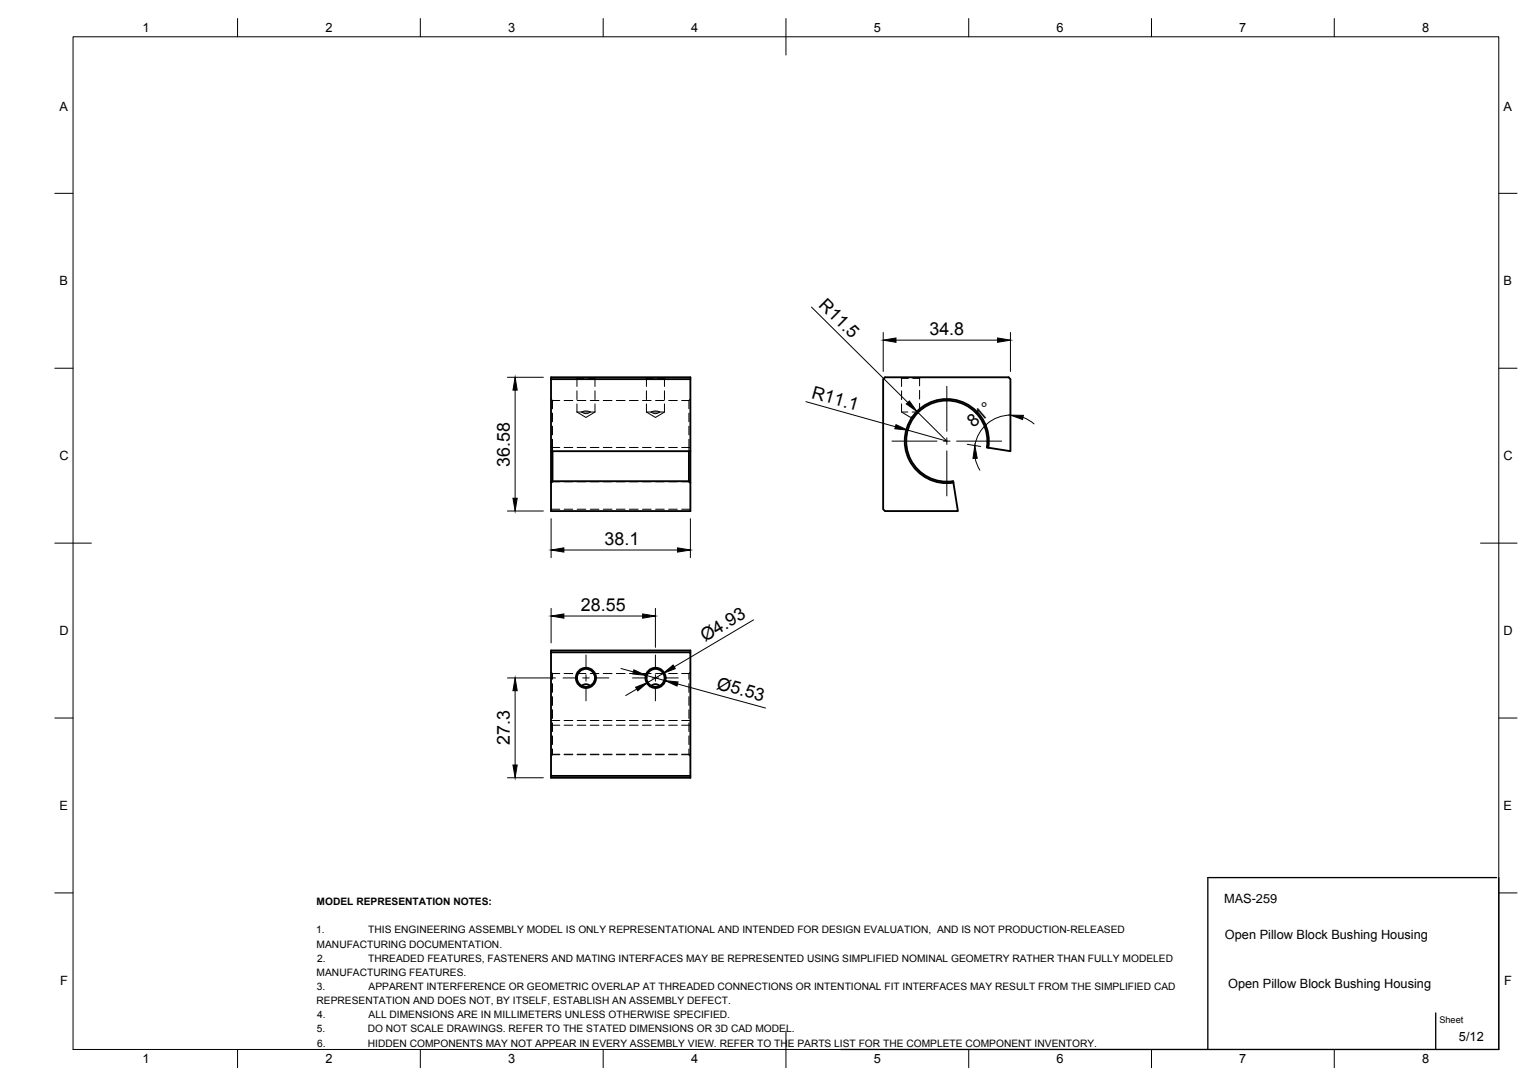
ISO-10303-21;
HEADER;
/* Generated by software containing ST-Developer
 * from STEP Tools, Inc. (www.steptools.com) 
 */

FILE_DESCRIPTION(
/* description */ (''),
/* implementation_level */ '2;1');

FILE_NAME(
/* name */ 'Open Pillow Block Bushing Housing.step',
/* time_stamp */ '2026-10-15T13:30:17-07:00',
/* author */ (''),
/* organization */ (''),
/* preprocessor_version */ 'ST-DEVELOPER v20.2',
/* originating_system */ 'Autodesk Translation Framework v15.15.0.0',
/* authorisation */ '');

FILE_SCHEMA (('AUTOMOTIVE_DESIGN { 1 0 10303 214 3 1 1 }'));
ENDSEC;

DATA;
#10=MECHANICAL_DESIGN_GEOMETRIC_PRESENTATION_REPRESENTATION('',(#1036),#71795);
#1016=SHAPE_REPRESENTATION_RELATIONSHIP('SRR','None',#72020,#1026);
#1026=ADVANCED_BREP_SHAPE_REPRESENTATION('',(#1046),#71788);
#1036=STYLED_ITEM('',(#72079),#1046);
#1046=MANIFOLD_SOLID_BREP('Body1',#13638);
#1086=CONICAL_SURFACE('',#14013,2.61400000000001,0.785398163397456);
#1087=CONICAL_SURFACE('',#14021,2.61400000000001,0.785398163397456);
#1088=CONICAL_SURFACE('',#14026,2.464,1.02974425867666);
#1089=CONICAL_SURFACE('',#14030,2.464,1.02974425867665);
#1090=CONICAL_SURFACE('',#14031,11.3,0.785398163397451);
#1091=CONICAL_SURFACE('',#14035,11.3,0.785398163397451);
#1137=B_SPLINE_CURVE_WITH_KNOTS('',3,(#19561,#19562,#19563,#19564,#19565,
#19566,#19567,#19568,#19569,#19570,#19571,#19572,#19573,#19574),
 .UNSPECIFIED.,.F.,.F.,(4,2,2,2,2,2,4),(-1.14599907215265,-1.14082829651813,
-1.08169405294193,-1.02255980936573,-0.963425565789533,-0.904291322213332,
-0.899120546578817),.UNSPECIFIED.);
#1138=B_SPLINE_CURVE_WITH_KNOTS('',3,(#19586,#19587,#19588,#19589,#19590,
#19591,#19592,#19593,#19594,#19595,#19596,#19597,#19598,#19599),
 .UNSPECIFIED.,.F.,.F.,(4,2,2,2,2,2,4),(-1.14599907215265,-1.14082829651813,
-1.08169405294193,-1.02255980936573,-0.963425565789533,-0.904291322213332,
-0.899120546578816),.UNSPECIFIED.);
#1139=B_SPLINE_CURVE_WITH_KNOTS('',3,(#19604,#19605,#19606,#19607,#19608,
#19609,#19610,#19611,#19612,#19613,#19614,#19615,#19616,#19617),
 .UNSPECIFIED.,.F.,.F.,(4,2,2,2,2,2,4),(-0.440637337632516,-0.41817718819756,
-0.36956984330978,-0.309581883490714,-0.249593923671647,-0.200986578783867,
-0.178526429348912),.UNSPECIFIED.);
#1140=B_SPLINE_CURVE_WITH_KNOTS('',3,(#19627,#19628,#19629,#19630,#19631,
#19632,#19633,#19634,#19635,#19636,#19637,#19638,#19639,#19640),
 .UNSPECIFIED.,.F.,.F.,(4,2,2,2,2,2,4),(0.787224364416541,0.851680919549612,
0.89358137447704,0.935481829404467,0.977382284331895,1.01928273925932,1.08373929439239),
 .UNSPECIFIED.);
#1545=FACE_BOUND('',#2869,.T.);
#1546=FACE_BOUND('',#2870,.T.);
#1547=FACE_BOUND('',#2876,.T.);
#1548=FACE_BOUND('',#2877,.T.);
#1613=PLANE('',#14016);
#1614=PLANE('',#14033);
#1615=PLANE('',#14034);
#1616=PLANE('',#14037);
#1617=PLANE('',#14038);
#1618=PLANE('',#14039);
#1619=PLANE('',#14040);
#1620=PLANE('',#14041);
#1621=PLANE('',#14042);
#1622=PLANE('',#14043);
#1623=PLANE('',#14044);
#2158=FACE_OUTER_BOUND('',#2867,.T.);
#2159=FACE_OUTER_BOUND('',#2868,.T.);
#2160=FACE_OUTER_BOUND('',#2871,.T.);
#2161=FACE_OUTER_BOUND('',#2872,.T.);
#2162=FACE_OUTER_BOUND('',#2873,.T.);
#2163=FACE_OUTER_BOUND('',#2874,.T.);
#2164=FACE_OUTER_BOUND('',#2875,.T.);
#2165=FACE_OUTER_BOUND('',#2878,.T.);
#2166=FACE_OUTER_BOUND('',#2879,.T.);
#2167=FACE_OUTER_BOUND('',#2880,.T.);
#2168=FACE_OUTER_BOUND('',#2881,.T.);
#2169=FACE_OUTER_BOUND('',#2882,.T.);
#2170=FACE_OUTER_BOUND('',#2883,.T.);
#2171=FACE_OUTER_BOUND('',#2884,.T.);
#2172=FACE_OUTER_BOUND('',#2885,.T.);
#2173=FACE_OUTER_BOUND('',#2886,.T.);
#2174=FACE_OUTER_BOUND('',#2887,.T.);
#2175=FACE_OUTER_BOUND('',#2888,.T.);
#2176=FACE_OUTER_BOUND('',#2889,.T.);
#2177=FACE_OUTER_BOUND('',#2890,.T.);
#2867=EDGE_LOOP('',(#9569,#9570,#9571,#9572));
#2868=EDGE_LOOP('',(#9573,#9574,#9575,#9576));
#2869=EDGE_LOOP('',(#9577));
#2870=EDGE_LOOP('',(#9578));
#2871=EDGE_LOOP('',(#9579,#9580,#9581,#9582,#9583,#9584));
#2872=EDGE_LOOP('',(#9585,#9586,#9587,#9588));
#2873=EDGE_LOOP('',(#9589,#9590,#9591,#9592,#9593,#9594));
#2874=EDGE_LOOP('',(#9595,#9596,#9597,#9598,#9599));
#2875=EDGE_LOOP('',(#9600,#9601,#9602,#9603));
#2876=EDGE_LOOP('',(#9604,#9605));
#2877=EDGE_LOOP('',(#9606,#9607));
#2878=EDGE_LOOP('',(#9608,#9609,#9610,#9611,#9612));
#2879=EDGE_LOOP('',(#9613,#9614,#9615,#9616));
#2880=EDGE_LOOP('',(#9617,#9618,#9619,#9620,#9621,#9622,#9623,#9624,#9625,
#9626));
#2881=EDGE_LOOP('',(#9627,#9628,#9629,#9630,#9631,#9632));
#2882=EDGE_LOOP('',(#9633,#9634,#9635,#9636));
#2883=EDGE_LOOP('',(#9637,#9638,#9639,#9640,#9641,#9642,#9643,#9644,#9645,
#9646));
#2884=EDGE_LOOP('',(#9647,#9648,#9649,#9650,#9651,#9652));
#2885=EDGE_LOOP('',(#9653,#9654,#9655,#9656));
#2886=EDGE_LOOP('',(#9657,#9658,#9659,#9660));
#2887=EDGE_LOOP('',(#9661,#9662,#9663,#9664));
#2888=EDGE_LOOP('',(#9665,#9666,#9667,#9668));
#2889=EDGE_LOOP('',(#9669,#9670,#9671,#9672));
#2890=EDGE_LOOP('',(#9673,#9674,#9675,#9676));
#3519=CIRCLE('',#14014,2.464);
#3520=CIRCLE('',#14015,2.76400000000001);
#3521=CIRCLE('',#14017,2.76400000000001);
#3522=CIRCLE('',#14019,2.464);
#3523=CIRCLE('',#14020,2.464);
#3524=CIRCLE('',#14022,2.464);
#3525=CIRCLE('',#14024,2.464);
#3526=CIRCLE('',#14025,2.464);
#3527=CIRCLE('',#14028,11.1);
#3528=CIRCLE('',#14029,11.1);
#3529=CIRCLE('',#14032,11.5);
#3530=CIRCLE('',#14036,11.5);
#3985=LINE('',#19542,#4896);
#3986=LINE('',#19547,#4897);
#3987=LINE('',#19549,#4898);
#3988=LINE('',#19551,#4899);
#3989=LINE('',#19552,#4900);
#3990=LINE('',#19557,#4901);
#3991=LINE('',#19579,#4902);
#3992=LINE('',#19582,#4903);
#3993=LINE('',#19603,#4904);
#3994=LINE('',#19623,#4905);
#3995=LINE('',#19626,#4906);
#3996=LINE('',#19643,#4907);
#3997=LINE('',#19646,#4908);
#3998=LINE('',#19649,#4909);
#3999=LINE('',#19652,#4910);
#4000=LINE('',#19654,#4911);
#4001=LINE('',#19655,#4912);
#4002=LINE('',#19657,#4913);
#4003=LINE('',#19659,#4914);
#4004=LINE('',#19661,#4915);
#4005=LINE('',#19663,#4916);
#4006=LINE('',#19664,#4917);
#4007=LINE('',#19667,#4918);
#4008=LINE('',#19669,#4919);
#4009=LINE('',#19670,#4920);
#4010=LINE('',#19673,#4921);
#4011=LINE('',#19677,#4922);
#4012=LINE('',#19679,#4923);
#4013=LINE('',#19681,#4924);
#4014=LINE('',#19683,#4925);
#4015=LINE('',#19684,#4926);
#4016=LINE('',#19686,#4927);
#4017=LINE('',#19687,#4928);
#4018=LINE('',#19689,#4929);
#4019=LINE('',#19691,#4930);
#4020=LINE('',#19693,#4931);
#4021=LINE('',#19695,#4932);
#4022=LINE('',#19697,#4933);
#4896=VECTOR('',#15708,2.61400000000001);
#4897=VECTOR('',#15713,10.);
#4898=VECTOR('',#15714,10.);
#4899=VECTOR('',#15715,10.);
#4900=VECTOR('',#15716,10.);
#4901=VECTOR('',#15721,2.464);
#4902=VECTOR('',#15730,2.61400000000001);
#4903=VECTOR('',#15733,2.464);
#4904=VECTOR('',#15740,2.464);
#4905=VECTOR('',#15745,10.);
#4906=VECTOR('',#15748,10.);
#4907=VECTOR('',#15751,2.464);
#4908=VECTOR('',#15754,10.);
#4909=VECTOR('',#15757,10.);
#4910=VECTOR('',#15760,10.);
#4911=VECTOR('',#15761,10.);
#4912=VECTOR('',#15762,10.);
#4913=VECTOR('',#15763,10.);
#4914=VECTOR('',#15764,10.);
#4915=VECTOR('',#15765,10.);
#4916=VECTOR('',#15766,10.);
#4917=VECTOR('',#15767,10.);
#4918=VECTOR('',#15770,10.);
#4919=VECTOR('',#15771,10.);
#4920=VECTOR('',#15772,10.);
#4921=VECTOR('',#15775,10.);
#4922=VECTOR('',#15780,10.);
#4923=VECTOR('',#15781,10.);
#4924=VECTOR('',#15782,10.);
#4925=VECTOR('',#15783,10.);
#4926=VECTOR('',#15784,10.);
#4927=VECTOR('',#15785,10.);
#4928=VECTOR('',#15786,10.);
#4929=VECTOR('',#15789,10.);
#4930=VECTOR('',#15792,10.);
#4931=VECTOR('',#15795,10.);
#4932=VECTOR('',#15798,10.);
#4933=VECTOR('',#15801,10.);
#5868=VERTEX_POINT('',#19539);
#5869=VERTEX_POINT('',#19541);
#5870=VERTEX_POINT('',#19545);
#5871=VERTEX_POINT('',#19546);
#5872=VERTEX_POINT('',#19548);
#5873=VERTEX_POINT('',#19550);
#5874=VERTEX_POINT('',#19553);
#5875=VERTEX_POINT('',#19556);
#5876=VERTEX_POINT('',#19558);
#5877=VERTEX_POINT('',#19560);
#5878=VERTEX_POINT('',#19577);
#5879=VERTEX_POINT('',#19581);
#5880=VERTEX_POINT('',#19583);
#5881=VERTEX_POINT('',#19585);
#5882=VERTEX_POINT('',#19602);
#5883=VERTEX_POINT('',#19619);
#5884=VERTEX_POINT('',#19620);
#5885=VERTEX_POINT('',#19622);
#5886=VERTEX_POINT('',#19624);
#5887=VERTEX_POINT('',#19642);
#5888=VERTEX_POINT('',#19645);
#5889=VERTEX_POINT('',#19647);
#5890=VERTEX_POINT('',#19651);
#5891=VERTEX_POINT('',#19653);
#5892=VERTEX_POINT('',#19656);
#5893=VERTEX_POINT('',#19658);
#5894=VERTEX_POINT('',#19660);
#5895=VERTEX_POINT('',#19662);
#5896=VERTEX_POINT('',#19666);
#5897=VERTEX_POINT('',#19668);
#5898=VERTEX_POINT('',#19672);
#5899=VERTEX_POINT('',#19676);
#5900=VERTEX_POINT('',#19678);
#5901=VERTEX_POINT('',#19680);
#5902=VERTEX_POINT('',#19682);
#5903=VERTEX_POINT('',#19685);
#7319=EDGE_CURVE('',#5868,#5868,#3519,.T.);
#7320=EDGE_CURVE('',#5868,#5869,#3985,.T.);
#7321=EDGE_CURVE('',#5869,#5869,#3520,.T.);
#7322=EDGE_CURVE('',#5870,#5871,#3986,.T.);
#7323=EDGE_CURVE('',#5872,#5870,#3987,.T.);
#7324=EDGE_CURVE('',#5873,#5872,#3988,.T.);
#7325=EDGE_CURVE('',#5871,#5873,#3989,.T.);
#7326=EDGE_CURVE('',#5874,#5874,#3521,.T.);
#7327=EDGE_CURVE('',#5868,#5875,#3990,.T.);
#7328=EDGE_CURVE('',#5875,#5876,#3522,.T.);
#7329=EDGE_CURVE('',#5877,#5876,#1137,.T.);
#7330=EDGE_CURVE('',#5877,#5875,#3523,.T.);
#7331=EDGE_CURVE('',#5878,#5878,#3524,.T.);
#7332=EDGE_CURVE('',#5878,#5874,#3991,.T.);
#7333=EDGE_CURVE('',#5878,#5879,#3992,.T.);
#7334=EDGE_CURVE('',#5879,#5880,#3525,.T.);
#7335=EDGE_CURVE('',#5881,#5880,#1138,.T.);
#7336=EDGE_CURVE('',#5881,#5879,#3526,.T.);
#7337=EDGE_CURVE('',#5882,#5875,#3993,.T.);
#7338=EDGE_CURVE('',#5876,#5877,#1139,.T.);
#7339=EDGE_CURVE('',#5883,#5884,#3527,.T.);
#7340=EDGE_CURVE('',#5885,#5883,#3994,.T.);
#7341=EDGE_CURVE('',#5886,#5885,#3528,.T.);
#7342=EDGE_CURVE('',#5884,#5886,#3995,.T.);
#7343=EDGE_CURVE('',#5880,#5881,#1140,.T.);
#7344=EDGE_CURVE('',#5887,#5879,#3996,.T.);
#7345=EDGE_CURVE('',#5884,#5888,#3997,.T.);
#7346=EDGE_CURVE('',#5888,#5889,#3529,.T.);
#7347=EDGE_CURVE('',#5889,#5883,#3998,.T.);
#7348=EDGE_CURVE('',#5888,#5890,#3999,.T.);
#7349=EDGE_CURVE('',#5890,#5891,#4000,.T.);
#7350=EDGE_CURVE('',#5871,#5891,#4001,.T.);
#7351=EDGE_CURVE('',#5892,#5873,#4002,.T.);
#7352=EDGE_CURVE('',#5892,#5893,#4003,.T.);
#7353=EDGE_CURVE('',#5894,#5893,#4004,.T.);
#7354=EDGE_CURVE('',#5894,#5895,#4005,.T.);
#7355=EDGE_CURVE('',#5895,#5889,#4006,.T.);
#7356=EDGE_CURVE('',#5896,#5886,#4007,.T.);
#7357=EDGE_CURVE('',#5897,#5896,#4008,.T.);
#7358=EDGE_CURVE('',#5897,#5890,#4009,.T.);
#7359=EDGE_CURVE('',#5885,#5898,#4010,.T.);
#7360=EDGE_CURVE('',#5898,#5896,#3530,.T.);
#7361=EDGE_CURVE('',#5898,#5899,#4011,.T.);
#7362=EDGE_CURVE('',#5899,#5900,#4012,.T.);
#7363=EDGE_CURVE('',#5901,#5900,#4013,.T.);
#7364=EDGE_CURVE('',#5901,#5902,#4014,.T.);
#7365=EDGE_CURVE('',#5872,#5902,#4015,.T.);
#7366=EDGE_CURVE('',#5903,#5870,#4016,.T.);
#7367=EDGE_CURVE('',#5903,#5897,#4017,.T.);
#7368=EDGE_CURVE('',#5899,#5895,#4018,.T.);
#7369=EDGE_CURVE('',#5891,#5903,#4019,.T.);
#7370=EDGE_CURVE('',#5902,#5892,#4020,.T.);
#7371=EDGE_CURVE('',#5893,#5901,#4021,.T.);
#7372=EDGE_CURVE('',#5900,#5894,#4022,.T.);
#9569=ORIENTED_EDGE('',*,*,#7319,.T.);
#9570=ORIENTED_EDGE('',*,*,#7320,.T.);
#9571=ORIENTED_EDGE('',*,*,#7321,.T.);
#9572=ORIENTED_EDGE('',*,*,#7320,.F.);
#9573=ORIENTED_EDGE('',*,*,#7322,.F.);
#9574=ORIENTED_EDGE('',*,*,#7323,.F.);
#9575=ORIENTED_EDGE('',*,*,#7324,.F.);
#9576=ORIENTED_EDGE('',*,*,#7325,.F.);
#9577=ORIENTED_EDGE('',*,*,#7326,.F.);
#9578=ORIENTED_EDGE('',*,*,#7321,.F.);
#9579=ORIENTED_EDGE('',*,*,#7319,.F.);
#9580=ORIENTED_EDGE('',*,*,#7327,.T.);
#9581=ORIENTED_EDGE('',*,*,#7328,.T.);
#9582=ORIENTED_EDGE('',*,*,#7329,.F.);
#9583=ORIENTED_EDGE('',*,*,#7330,.T.);
#9584=ORIENTED_EDGE('',*,*,#7327,.F.);
#9585=ORIENTED_EDGE('',*,*,#7331,.T.);
#9586=ORIENTED_EDGE('',*,*,#7332,.T.);
#9587=ORIENTED_EDGE('',*,*,#7326,.T.);
#9588=ORIENTED_EDGE('',*,*,#7332,.F.);
#9589=ORIENTED_EDGE('',*,*,#7331,.F.);
#9590=ORIENTED_EDGE('',*,*,#7333,.T.);
#9591=ORIENTED_EDGE('',*,*,#7334,.T.);
#9592=ORIENTED_EDGE('',*,*,#7335,.F.);
#9593=ORIENTED_EDGE('',*,*,#7336,.T.);
#9594=ORIENTED_EDGE('',*,*,#7333,.F.);
#9595=ORIENTED_EDGE('',*,*,#7337,.T.);
#9596=ORIENTED_EDGE('',*,*,#7330,.F.);
#9597=ORIENTED_EDGE('',*,*,#7338,.F.);
#9598=ORIENTED_EDGE('',*,*,#7328,.F.);
#9599=ORIENTED_EDGE('',*,*,#7337,.F.);
#9600=ORIENTED_EDGE('',*,*,#7339,.F.);
#9601=ORIENTED_EDGE('',*,*,#7340,.F.);
#9602=ORIENTED_EDGE('',*,*,#7341,.F.);
#9603=ORIENTED_EDGE('',*,*,#7342,.F.);
#9604=ORIENTED_EDGE('',*,*,#7343,.T.);
#9605=ORIENTED_EDGE('',*,*,#7335,.T.);
#9606=ORIENTED_EDGE('',*,*,#7338,.T.);
#9607=ORIENTED_EDGE('',*,*,#7329,.T.);
#9608=ORIENTED_EDGE('',*,*,#7344,.T.);
#9609=ORIENTED_EDGE('',*,*,#7336,.F.);
#9610=ORIENTED_EDGE('',*,*,#7343,.F.);
#9611=ORIENTED_EDGE('',*,*,#7334,.F.);
#9612=ORIENTED_EDGE('',*,*,#7344,.F.);
#9613=ORIENTED_EDGE('',*,*,#7345,.T.);
#9614=ORIENTED_EDGE('',*,*,#7346,.T.);
#9615=ORIENTED_EDGE('',*,*,#7347,.T.);
#9616=ORIENTED_EDGE('',*,*,#7339,.T.);
#9617=ORIENTED_EDGE('',*,*,#7346,.F.);
#9618=ORIENTED_EDGE('',*,*,#7348,.T.);
#9619=ORIENTED_EDGE('',*,*,#7349,.T.);
#9620=ORIENTED_EDGE('',*,*,#7350,.F.);
#9621=ORIENTED_EDGE('',*,*,#7325,.T.);
#9622=ORIENTED_EDGE('',*,*,#7351,.F.);
#9623=ORIENTED_EDGE('',*,*,#7352,.T.);
#9624=ORIENTED_EDGE('',*,*,#7353,.F.);
#9625=ORIENTED_EDGE('',*,*,#7354,.T.);
#9626=ORIENTED_EDGE('',*,*,#7355,.T.);
#9627=ORIENTED_EDGE('',*,*,#7345,.F.);
#9628=ORIENTED_EDGE('',*,*,#7342,.T.);
#9629=ORIENTED_EDGE('',*,*,#7356,.F.);
#9630=ORIENTED_EDGE('',*,*,#7357,.F.);
#9631=ORIENTED_EDGE('',*,*,#7358,.T.);
#9632=ORIENTED_EDGE('',*,*,#7348,.F.);
#9633=ORIENTED_EDGE('',*,*,#7359,.T.);
#9634=ORIENTED_EDGE('',*,*,#7360,.T.);
#9635=ORIENTED_EDGE('',*,*,#7356,.T.);
#9636=ORIENTED_EDGE('',*,*,#7341,.T.);
#9637=ORIENTED_EDGE('',*,*,#7360,.F.);
#9638=ORIENTED_EDGE('',*,*,#7361,.T.);
#9639=ORIENTED_EDGE('',*,*,#7362,.T.);
#9640=ORIENTED_EDGE('',*,*,#7363,.F.);
#9641=ORIENTED_EDGE('',*,*,#7364,.T.);
#9642=ORIENTED_EDGE('',*,*,#7365,.F.);
#9643=ORIENTED_EDGE('',*,*,#7323,.T.);
#9644=ORIENTED_EDGE('',*,*,#7366,.F.);
#9645=ORIENTED_EDGE('',*,*,#7367,.T.);
#9646=ORIENTED_EDGE('',*,*,#7357,.T.);
#9647=ORIENTED_EDGE('',*,*,#7347,.F.);
#9648=ORIENTED_EDGE('',*,*,#7355,.F.);
#9649=ORIENTED_EDGE('',*,*,#7368,.F.);
#9650=ORIENTED_EDGE('',*,*,#7361,.F.);
#9651=ORIENTED_EDGE('',*,*,#7359,.F.);
#9652=ORIENTED_EDGE('',*,*,#7340,.T.);
#9653=ORIENTED_EDGE('',*,*,#7350,.T.);
#9654=ORIENTED_EDGE('',*,*,#7369,.T.);
#9655=ORIENTED_EDGE('',*,*,#7366,.T.);
#9656=ORIENTED_EDGE('',*,*,#7322,.T.);
#9657=ORIENTED_EDGE('',*,*,#7351,.T.);
#9658=ORIENTED_EDGE('',*,*,#7324,.T.);
#9659=ORIENTED_EDGE('',*,*,#7365,.T.);
#9660=ORIENTED_EDGE('',*,*,#7370,.T.);
#9661=ORIENTED_EDGE('',*,*,#7370,.F.);
#9662=ORIENTED_EDGE('',*,*,#7364,.F.);
#9663=ORIENTED_EDGE('',*,*,#7371,.F.);
#9664=ORIENTED_EDGE('',*,*,#7352,.F.);
#9665=ORIENTED_EDGE('',*,*,#7353,.T.);
#9666=ORIENTED_EDGE('',*,*,#7371,.T.);
#9667=ORIENTED_EDGE('',*,*,#7363,.T.);
#9668=ORIENTED_EDGE('',*,*,#7372,.T.);
#9669=ORIENTED_EDGE('',*,*,#7372,.F.);
#9670=ORIENTED_EDGE('',*,*,#7362,.F.);
#9671=ORIENTED_EDGE('',*,*,#7368,.T.);
#9672=ORIENTED_EDGE('',*,*,#7354,.F.);
#9673=ORIENTED_EDGE('',*,*,#7369,.F.);
#9674=ORIENTED_EDGE('',*,*,#7349,.F.);
#9675=ORIENTED_EDGE('',*,*,#7358,.F.);
#9676=ORIENTED_EDGE('',*,*,#7367,.F.);
#12911=CYLINDRICAL_SURFACE('',#14018,2.464);
#12912=CYLINDRICAL_SURFACE('',#14023,2.464);
#12913=CYLINDRICAL_SURFACE('',#14027,11.1);
#13118=ADVANCED_FACE('',(#2158),#1086,.F.);
#13119=ADVANCED_FACE('',(#2159,#1545,#1546),#1613,.T.);
#13120=ADVANCED_FACE('',(#2160),#12911,.F.);
#13121=ADVANCED_FACE('',(#2161),#1087,.F.);
#13122=ADVANCED_FACE('',(#2162),#12912,.F.);
#13123=ADVANCED_FACE('',(#2163),#1088,.F.);
#13124=ADVANCED_FACE('',(#2164,#1547,#1548),#12913,.F.);
#13125=ADVANCED_FACE('',(#2165),#1089,.F.);
#13126=ADVANCED_FACE('',(#2166),#1090,.F.);
#13127=ADVANCED_FACE('',(#2167),#1614,.T.);
#13128=ADVANCED_FACE('',(#2168),#1615,.T.);
#13129=ADVANCED_FACE('',(#2169),#1091,.F.);
#13130=ADVANCED_FACE('',(#2170),#1616,.F.);
#13131=ADVANCED_FACE('',(#2171),#1617,.T.);
#13132=ADVANCED_FACE('',(#2172),#1618,.T.);
#13133=ADVANCED_FACE('',(#2173),#1619,.T.);
#13134=ADVANCED_FACE('',(#2174),#1620,.T.);
#13135=ADVANCED_FACE('',(#2175),#1621,.T.);
#13136=ADVANCED_FACE('',(#2176),#1622,.T.);
#13137=ADVANCED_FACE('',(#2177),#1623,.T.);
#13638=CLOSED_SHELL('',(#13118,#13119,#13120,#13121,#13122,#13123,#13124,
#13125,#13126,#13127,#13128,#13129,#13130,#13131,#13132,#13133,#13134,#13135,
#13136,#13137));
#14012=AXIS2_PLACEMENT_3D('',#19537,#15702,#15703);
#14013=AXIS2_PLACEMENT_3D('',#19538,#15704,#15705);
#14014=AXIS2_PLACEMENT_3D('',#19540,#15706,#15707);
#14015=AXIS2_PLACEMENT_3D('',#19543,#15709,#15710);
#14016=AXIS2_PLACEMENT_3D('',#19544,#15711,#15712);
#14017=AXIS2_PLACEMENT_3D('',#19554,#15717,#15718);
#14018=AXIS2_PLACEMENT_3D('',#19555,#15719,#15720);
#14019=AXIS2_PLACEMENT_3D('',#19559,#15722,#15723);
#14020=AXIS2_PLACEMENT_3D('',#19575,#15724,#15725);
#14021=AXIS2_PLACEMENT_3D('',#19576,#15726,#15727);
#14022=AXIS2_PLACEMENT_3D('',#19578,#15728,#15729);
#14023=AXIS2_PLACEMENT_3D('',#19580,#15731,#15732);
#14024=AXIS2_PLACEMENT_3D('',#19584,#15734,#15735);
#14025=AXIS2_PLACEMENT_3D('',#19600,#15736,#15737);
#14026=AXIS2_PLACEMENT_3D('',#19601,#15738,#15739);
#14027=AXIS2_PLACEMENT_3D('',#19618,#15741,#15742);
#14028=AXIS2_PLACEMENT_3D('',#19621,#15743,#15744);
#14029=AXIS2_PLACEMENT_3D('',#19625,#15746,#15747);
#14030=AXIS2_PLACEMENT_3D('',#19641,#15749,#15750);
#14031=AXIS2_PLACEMENT_3D('',#19644,#15752,#15753);
#14032=AXIS2_PLACEMENT_3D('',#19648,#15755,#15756);
#14033=AXIS2_PLACEMENT_3D('',#19650,#15758,#15759);
#14034=AXIS2_PLACEMENT_3D('',#19665,#15768,#15769);
#14035=AXIS2_PLACEMENT_3D('',#19671,#15773,#15774);
#14036=AXIS2_PLACEMENT_3D('',#19674,#15776,#15777);
#14037=AXIS2_PLACEMENT_3D('',#19675,#15778,#15779);
#14038=AXIS2_PLACEMENT_3D('',#19688,#15787,#15788);
#14039=AXIS2_PLACEMENT_3D('',#19690,#15790,#15791);
#14040=AXIS2_PLACEMENT_3D('',#19692,#15793,#15794);
#14041=AXIS2_PLACEMENT_3D('',#19694,#15796,#15797);
#14042=AXIS2_PLACEMENT_3D('',#19696,#15799,#15800);
#14043=AXIS2_PLACEMENT_3D('',#19698,#15802,#15803);
#14044=AXIS2_PLACEMENT_3D('',#19699,#15804,#15805);
#15702=DIRECTION('axis',(0.,0.,1.));
#15703=DIRECTION('refdir',(1.,0.,0.));
#15704=DIRECTION('center_axis',(0.,1.,0.));
#15705=DIRECTION('ref_axis',(1.,0.,0.));
#15706=DIRECTION('center_axis',(0.,-1.,0.));
#15707=DIRECTION('ref_axis',(1.,0.,0.));
#15708=DIRECTION('',(-0.707106781186553,0.707106781186542,8.659560562355E-17));
#15709=DIRECTION('center_axis',(0.,1.,0.));
#15710=DIRECTION('ref_axis',(1.,0.,0.));
#15711=DIRECTION('center_axis',(0.,1.,0.));
#15712=DIRECTION('ref_axis',(0.,0.,1.));
#15713=DIRECTION('',(1.,0.,0.));
#15714=DIRECTION('',(0.,0.,-1.));
#15715=DIRECTION('',(-1.,0.,0.));
#15716=DIRECTION('',(0.,0.,1.));
#15717=DIRECTION('center_axis',(0.,1.,0.));
#15718=DIRECTION('ref_axis',(1.,0.,0.));
#15719=DIRECTION('center_axis',(0.,-1.,0.));
#15720=DIRECTION('ref_axis',(1.,0.,0.));
#15721=DIRECTION('',(0.,-1.,0.));
#15722=DIRECTION('center_axis',(0.,-1.,0.));
#15723=DIRECTION('ref_axis',(1.,0.,0.));
#15724=DIRECTION('center_axis',(0.,-1.,0.));
#15725=DIRECTION('ref_axis',(1.,0.,0.));
#15726=DIRECTION('center_axis',(0.,1.,0.));
#15727=DIRECTION('ref_axis',(1.,0.,0.));
#15728=DIRECTION('center_axis',(0.,-1.,0.));
#15729=DIRECTION('ref_axis',(1.,0.,0.));
#15730=DIRECTION('',(-0.707106781186553,0.707106781186542,8.659560562355E-17));
#15731=DIRECTION('center_axis',(0.,-1.,0.));
#15732=DIRECTION('ref_axis',(1.,0.,0.));
#15733=DIRECTION('',(0.,-1.,0.));
#15734=DIRECTION('center_axis',(0.,-1.,0.));
#15735=DIRECTION('ref_axis',(1.,0.,0.));
#15736=DIRECTION('center_axis',(0.,-1.,0.));
#15737=DIRECTION('ref_axis',(1.,0.,0.));
#15738=DIRECTION('center_axis',(0.,1.,0.));
#15739=DIRECTION('ref_axis',(1.,0.,0.));
#15740=DIRECTION('',(-0.857167300702115,0.515038074910049,1.04972719113862E-16));
#15741=DIRECTION('center_axis',(1.,0.,0.));
#15742=DIRECTION('ref_axis',(0.,0.707106781186547,0.707106781186547));
#15743=DIRECTION('center_axis',(-1.,0.,0.));
#15744=DIRECTION('ref_axis',(0.,0.,1.));
#15745=DIRECTION('',(1.,0.,0.));
#15746=DIRECTION('center_axis',(1.,0.,0.));
#15747=DIRECTION('ref_axis',(0.,0.,1.));
#15748=DIRECTION('',(-1.,0.,0.));
#15749=DIRECTION('center_axis',(0.,1.,0.));
#15750=DIRECTION('ref_axis',(1.,0.,0.));
#15751=DIRECTION('',(-0.85716730070211,0.515038074910058,1.04972719113862E-16));
#15752=DIRECTION('center_axis',(1.,0.,0.));
#15753=DIRECTION('ref_axis',(0.,0.707106781186547,0.707106781186548));
#15754=DIRECTION('',(0.707106781186546,-0.110615871041237,-0.698401123333712));
#15755=DIRECTION('center_axis',(1.,0.,0.));
#15756=DIRECTION('ref_axis',(0.,0.,1.));
#15757=DIRECTION('',(-0.707106781186546,0.698401123333712,0.110615871041237));
#15758=DIRECTION('center_axis',(1.,0.,0.));
#15759=DIRECTION('ref_axis',(0.,0.,-1.));
#15760=DIRECTION('',(0.,-0.156434465040231,-0.987688340595138));
#15761=DIRECTION('',(0.,1.,0.));
#15762=DIRECTION('',(0.,-0.707106781186547,-0.707106781186547));
#15763=DIRECTION('',(0.,0.707106781186547,-0.707106781186547));
#15764=DIRECTION('',(0.,-1.,0.));
#15765=DIRECTION('',(0.,0.707106781186543,0.707106781186552));
#15766=DIRECTION('',(0.,0.,-1.));
#15767=DIRECTION('',(0.,0.987688340595138,0.156434465040231));
#15768=DIRECTION('center_axis',(0.,-0.987688340595138,0.156434465040231));
#15769=DIRECTION('ref_axis',(0.,-0.156434465040231,-0.987688340595138));
#15770=DIRECTION('',(0.707106781186546,0.110615871041237,0.698401123333712));
#15771=DIRECTION('',(0.,0.156434465040231,0.987688340595138));
#15772=DIRECTION('',(1.,0.,0.));
#15773=DIRECTION('center_axis',(-1.,0.,0.));
#15774=DIRECTION('ref_axis',(0.,0.707106781186547,0.707106781186548));
#15775=DIRECTION('',(-0.707106781186546,-0.698401123333712,-0.110615871041237));
#15776=DIRECTION('center_axis',(-1.,0.,0.));
#15777=DIRECTION('ref_axis',(0.,0.,1.));
#15778=DIRECTION('center_axis',(1.,0.,0.));
#15779=DIRECTION('ref_axis',(0.,0.,-1.));
#15780=DIRECTION('',(0.,-0.987688340595138,-0.156434465040231));
#15781=DIRECTION('',(0.,0.,1.));
#15782=DIRECTION('',(0.,-0.707106781186543,-0.707106781186552));
#15783=DIRECTION('',(0.,1.,0.));
#15784=DIRECTION('',(0.,-0.707106781186547,0.707106781186547));
#15785=DIRECTION('',(0.,0.707106781186547,0.707106781186547));
#15786=DIRECTION('',(0.,-1.,0.));
#15787=DIRECTION('center_axis',(0.,0.156434465040231,-0.987688340595138));
#15788=DIRECTION('ref_axis',(0.,0.987688340595138,0.156434465040231));
#15789=DIRECTION('',(1.,0.,0.));
#15790=DIRECTION('center_axis',(0.,0.707106781186548,-0.707106781186548));
#15791=DIRECTION('ref_axis',(-1.,0.,0.));
#15792=DIRECTION('',(-1.,0.,0.));
#15793=DIRECTION('center_axis',(0.,0.707106781186548,0.707106781186548));
#15794=DIRECTION('ref_axis',(1.,0.,0.));
#15795=DIRECTION('',(1.,0.,0.));
#15796=DIRECTION('center_axis',(0.,0.,1.));
#15797=DIRECTION('ref_axis',(0.,-1.,0.));
#15798=DIRECTION('',(-1.,0.,0.));
#15799=DIRECTION('center_axis',(0.,-0.707106781186552,0.707106781186543));
#15800=DIRECTION('ref_axis',(1.,0.,0.));
#15801=DIRECTION('',(1.,0.,0.));
#15802=DIRECTION('center_axis',(0.,-1.,0.));
#15803=DIRECTION('ref_axis',(0.,0.,-1.));
#15804=DIRECTION('center_axis',(0.,0.,-1.));
#15805=DIRECTION('ref_axis',(0.,1.,0.));
#19537=CARTESIAN_POINT('',(0.,0.,0.));
#19538=CARTESIAN_POINT('Origin',(61.4,39.5248,48.));
#19539=CARTESIAN_POINT('',(58.936,39.3748,48.));
#19540=CARTESIAN_POINT('Origin',(61.4,39.3748,48.));
#19541=CARTESIAN_POINT('',(58.636,39.6748,48.));
#19542=CARTESIAN_POINT('',(58.786,39.5248,48.));
#19543=CARTESIAN_POINT('Origin',(61.4,39.6748,48.));
#19544=CARTESIAN_POINT('Origin',(32.85,39.6748,20.7));
#19545=CARTESIAN_POINT('',(32.85,39.6748,21.2));
#19546=CARTESIAN_POINT('',(70.95,39.6748,21.2));
#19547=CARTESIAN_POINT('',(32.85,39.6748,21.2));
#19548=CARTESIAN_POINT('',(32.85,39.6748,54.999));
#19549=CARTESIAN_POINT('',(32.85,39.6748,55.499));
#19550=CARTESIAN_POINT('',(70.95,39.6748,54.999));
#19551=CARTESIAN_POINT('',(32.85,39.6748,54.999));
#19552=CARTESIAN_POINT('',(70.95,39.6748,55.499));
#19553=CARTESIAN_POINT('',(39.636,39.6748,48.));
#19554=CARTESIAN_POINT('Origin',(42.4,39.6748,48.));
#19555=CARTESIAN_POINT('Origin',(61.4,39.6748,48.));
#19556=CARTESIAN_POINT('',(58.936,30.1748,48.));
#19557=CARTESIAN_POINT('',(58.936,39.6748,48.));
#19558=CARTESIAN_POINT('',(60.2023331707725,30.1748,45.8466560501935));
#19559=CARTESIAN_POINT('Origin',(61.4,30.1748,48.));
#19560=CARTESIAN_POINT('',(62.5976668292275,30.1748,45.8466560501935));
#19561=CARTESIAN_POINT('Ctrl Pts',(62.5976668292275,30.1748,45.8466560501935));
#19562=CARTESIAN_POINT('Ctrl Pts',(62.5839393404939,30.1822399802705,45.8390209680664));
#19563=CARTESIAN_POINT('Ctrl Pts',(62.5701440730763,30.1895277245944,45.8315201115594));
#19564=CARTESIAN_POINT('Ctrl Pts',(62.3978378742979,30.2782518989111,45.7399529520181));
#19565=CARTESIAN_POINT('Ctrl Pts',(62.2093398392196,30.3494894405534,45.6635629490944));
#19566=CARTESIAN_POINT('Ctrl Pts',(61.8090152862429,30.4433961447374,45.5614192720633));
#19567=CARTESIAN_POINT('Ctrl Pts',(61.597114145254,30.4661106047668,45.536));
#19568=CARTESIAN_POINT('Ctrl Pts',(61.202885854746,30.4661106047668,45.536));
#19569=CARTESIAN_POINT('Ctrl Pts',(60.9909847137571,30.4433961447374,45.5614192720633));
#19570=CARTESIAN_POINT('Ctrl Pts',(60.5906601607804,30.3494894405534,45.6635629490944));
#19571=CARTESIAN_POINT('Ctrl Pts',(60.4021621257021,30.2782518989111,45.7399529520181));
#19572=CARTESIAN_POINT('Ctrl Pts',(60.2298559269237,30.1895277245944,45.8315201115594));
#19573=CARTESIAN_POINT('Ctrl Pts',(60.2160606595061,30.1822399802704,45.8390209680664));
#19574=CARTESIAN_POINT('Ctrl Pts',(60.2023331707725,30.1748,45.8466560501935));
#19575=CARTESIAN_POINT('Origin',(61.4,30.1748,48.));
#19576=CARTESIAN_POINT('Origin',(42.4,39.5248,48.));
#19577=CARTESIAN_POINT('',(39.936,39.3748,48.));
#19578=CARTESIAN_POINT('Origin',(42.4,39.3748,48.));
#19579=CARTESIAN_POINT('',(39.786,39.5248,48.));
#19580=CARTESIAN_POINT('Origin',(42.4,39.6748,48.));
#19581=CARTESIAN_POINT('',(39.936,30.1748,48.));
#19582=CARTESIAN_POINT('',(39.936,39.6748,48.));
#19583=CARTESIAN_POINT('',(41.2023331707725,30.1748,45.8466560501935));
#19584=CARTESIAN_POINT('Origin',(42.4,30.1748,48.));
#19585=CARTESIAN_POINT('',(43.5976668292275,30.1748,45.8466560501935));
#19586=CARTESIAN_POINT('Ctrl Pts',(43.5976668292275,30.1748,45.8466560501935));
#19587=CARTESIAN_POINT('Ctrl Pts',(43.5839393404939,30.1822399802704,45.8390209680664));
#19588=CARTESIAN_POINT('Ctrl Pts',(43.5701440730763,30.1895277245944,45.8315201115594));
#19589=CARTESIAN_POINT('Ctrl Pts',(43.3978378742979,30.2782518989111,45.7399529520181));
#19590=CARTESIAN_POINT('Ctrl Pts',(43.2093398392196,30.3494894405534,45.6635629490944));
#19591=CARTESIAN_POINT('Ctrl Pts',(42.8090152862429,30.4433961447374,45.5614192720633));
#19592=CARTESIAN_POINT('Ctrl Pts',(42.597114145254,30.4661106047668,45.536));
#19593=CARTESIAN_POINT('Ctrl Pts',(42.202885854746,30.4661106047668,45.536));
#19594=CARTESIAN_POINT('Ctrl Pts',(41.9909847137571,30.4433961447374,45.5614192720633));
#19595=CARTESIAN_POINT('Ctrl Pts',(41.5906601607804,30.3494894405534,45.6635629490944));
#19596=CARTESIAN_POINT('Ctrl Pts',(41.4021621257021,30.2782518989111,45.7399529520181));
#19597=CARTESIAN_POINT('Ctrl Pts',(41.2298559269237,30.1895277245944,45.8315201115594));
#19598=CARTESIAN_POINT('Ctrl Pts',(41.216060659506,30.1822399802704,45.8390209680664));
#19599=CARTESIAN_POINT('Ctrl Pts',(41.2023331707725,30.1748,45.8466560501935));
#19600=CARTESIAN_POINT('Origin',(42.4,30.1748,48.));
#19601=CARTESIAN_POINT('Origin',(61.4,30.1748,48.));
#19602=CARTESIAN_POINT('',(61.4,28.6942794347161,48.));
#19603=CARTESIAN_POINT('',(58.936,30.1748,48.));
#19604=CARTESIAN_POINT('Ctrl Pts',(60.2023331707725,30.1748,45.8466560501935));
#19605=CARTESIAN_POINT('Ctrl Pts',(60.2597361109102,30.1384432612634,45.8839661875916));
#19606=CARTESIAN_POINT('Ctrl Pts',(60.3174608135473,30.1032893210344,45.9195148810763));
#19607=CARTESIAN_POINT('Ctrl Pts',(60.5005858709669,29.9969713807309,46.0257192203701));
#19608=CARTESIAN_POINT('Ctrl Pts',(60.6580928550894,29.9150369491545,46.1049725011069));
#19609=CARTESIAN_POINT('Ctrl Pts',(60.9740384574878,29.7867651942036,46.2264525494457));
#19610=CARTESIAN_POINT('Ctrl Pts',(61.2000401339365,29.7272527548782,46.2808436974387));
#19611=CARTESIAN_POINT('Ctrl Pts',(61.5999598660636,29.7272527548782,46.2808436974387));
#19612=CARTESIAN_POINT('Ctrl Pts',(61.8259615425122,29.7867651942036,46.2264525494457));
#19613=CARTESIAN_POINT('Ctrl Pts',(62.1419071449106,29.9150369491545,46.1049725011069));
#19614=CARTESIAN_POINT('Ctrl Pts',(62.2994141290331,29.9969713807309,46.0257192203701));
#19615=CARTESIAN_POINT('Ctrl Pts',(62.4825391864527,30.1032893210343,45.9195148810763));
#19616=CARTESIAN_POINT('Ctrl Pts',(62.5402638890898,30.1384432612634,45.8839661875916));
#19617=CARTESIAN_POINT('Ctrl Pts',(62.5976668292275,30.1748,45.8466560501935));
#19618=CARTESIAN_POINT('Origin',(32.85,22.225,38.1));
#19619=CARTESIAN_POINT('',(70.55,11.261659419394,36.3635774380534));
#19620=CARTESIAN_POINT('',(70.55,20.4885774380534,27.136659419394));
#19621=CARTESIAN_POINT('Origin',(70.55,22.225,38.1));
#19622=CARTESIAN_POINT('',(33.25,11.261659419394,36.3635774380534));
#19623=CARTESIAN_POINT('',(32.85,11.261659419394,36.3635774380534));
#19624=CARTESIAN_POINT('',(33.25,20.4885774380534,27.136659419394));
#19625=CARTESIAN_POINT('Origin',(33.25,22.225,38.1));
#19626=CARTESIAN_POINT('',(32.85,20.4885774380534,27.136659419394));
#19627=CARTESIAN_POINT('Ctrl Pts',(41.2023331707725,30.1748,45.8466560501935));
#19628=CARTESIAN_POINT('Ctrl Pts',(41.3584359963022,30.0759306802366,45.9481180633722));
#19629=CARTESIAN_POINT('Ctrl Pts',(41.5172853281954,29.9848847225031,46.0375998429581));
#19630=CARTESIAN_POINT('Ctrl Pts',(41.7909111977588,29.8583912347539,46.1589138702689));
#19631=CARTESIAN_POINT('Ctrl Pts',(41.9011722141917,29.8148256477821,46.1997866389185));
#19632=CARTESIAN_POINT('Ctrl Pts',(42.1359436639152,29.7493650522022,46.2606327740154));
#19633=CARTESIAN_POINT('Ctrl Pts',(42.2603318169086,29.7272527548782,46.2808436974387));
#19634=CARTESIAN_POINT('Ctrl Pts',(42.5396681830914,29.7272527548782,46.2808436974387));
#19635=CARTESIAN_POINT('Ctrl Pts',(42.6640563360848,29.7493650522022,46.2606327740154));
#19636=CARTESIAN_POINT('Ctrl Pts',(42.8988277858083,29.8148256477821,46.1997866389185));
#19637=CARTESIAN_POINT('Ctrl Pts',(43.0090888022412,29.8583912347539,46.1589138702689));
#19638=CARTESIAN_POINT('Ctrl Pts',(43.2827146718046,29.9848847225031,46.0375998429581));
#19639=CARTESIAN_POINT('Ctrl Pts',(43.4415640036978,30.0759306802366,45.9481180633722));
#19640=CARTESIAN_POINT('Ctrl Pts',(43.5976668292275,30.1748,45.8466560501935));
#19641=CARTESIAN_POINT('Origin',(42.4,30.1748,48.));
#19642=CARTESIAN_POINT('',(42.4,28.6942794347161,48.));
#19643=CARTESIAN_POINT('',(39.936,30.1748,48.));
#19644=CARTESIAN_POINT('Origin',(70.75,22.225,38.1));
#19645=CARTESIAN_POINT('',(70.95,20.4260036520373,26.7415840831559));
#19646=CARTESIAN_POINT('',(70.75,20.4572905450454,26.9391217512749));
#19647=CARTESIAN_POINT('',(70.95,10.8665840831559,36.3010036520373));
#19648=CARTESIAN_POINT('Origin',(70.95,22.225,38.1));
#19649=CARTESIAN_POINT('',(70.75,11.0641217512749,36.3322905450454));
#19650=CARTESIAN_POINT('Origin',(70.95,21.3868,38.0995));
#19651=CARTESIAN_POINT('',(70.95,19.4691107383531,20.7));
#19652=CARTESIAN_POINT('',(70.95,19.4691107383531,20.7));
#19653=CARTESIAN_POINT('',(70.95,39.1748,20.7));
#19654=CARTESIAN_POINT('',(70.95,39.6748,20.7));
#19655=CARTESIAN_POINT('',(70.95,39.202675,20.727875));
#19656=CARTESIAN_POINT('',(70.95,39.1748,55.499));
#19657=CARTESIAN_POINT('',(70.95,39.202675,55.471125));
#19658=CARTESIAN_POINT('',(70.95,3.5988,55.499));
#19659=CARTESIAN_POINT('',(70.95,3.0988,55.499));
#19660=CARTESIAN_POINT('',(70.95,3.0988,54.999));
#19661=CARTESIAN_POINT('',(70.95,3.57092499999994,55.4711249999999));
#19662=CARTESIAN_POINT('',(70.95,3.0988,35.0707075174648));
#19663=CARTESIAN_POINT('',(70.95,3.0988,35.0707075174648));
#19664=CARTESIAN_POINT('',(70.95,22.225,38.1));
#19665=CARTESIAN_POINT('Origin',(32.85,22.225,38.1));
#19666=CARTESIAN_POINT('',(32.85,20.4260036520373,26.7415840831559));
#19667=CARTESIAN_POINT('',(33.05,20.4572905450454,26.9391217512749));
#19668=CARTESIAN_POINT('',(32.85,19.4691107383531,20.7));
#19669=CARTESIAN_POINT('',(32.85,19.4691107383531,20.7));
#19670=CARTESIAN_POINT('',(32.85,19.4691107383531,20.7));
#19671=CARTESIAN_POINT('Origin',(33.05,22.225,38.1));
#19672=CARTESIAN_POINT('',(32.85,10.8665840831559,36.3010036520373));
#19673=CARTESIAN_POINT('',(33.05,11.0641217512749,36.3322905450454));
#19674=CARTESIAN_POINT('Origin',(32.85,22.225,38.1));
#19675=CARTESIAN_POINT('Origin',(32.85,21.3868,38.0995));
#19676=CARTESIAN_POINT('',(32.85,3.0988,35.0707075174648));
#19677=CARTESIAN_POINT('',(32.85,22.225,38.1));
#19678=CARTESIAN_POINT('',(32.85,3.0988,54.999));
#19679=CARTESIAN_POINT('',(32.85,3.0988,35.0707075174648));
#19680=CARTESIAN_POINT('',(32.85,3.5988,55.499));
#19681=CARTESIAN_POINT('',(32.85,3.57092499999994,55.4711249999999));
#19682=CARTESIAN_POINT('',(32.85,39.1748,55.499));
#19683=CARTESIAN_POINT('',(32.85,3.0988,55.499));
#19684=CARTESIAN_POINT('',(32.85,39.202675,55.471125));
#19685=CARTESIAN_POINT('',(32.85,39.1748,20.7));
#19686=CARTESIAN_POINT('',(32.85,39.202675,20.727875));
#19687=CARTESIAN_POINT('',(32.85,39.6748,20.7));
#19688=CARTESIAN_POINT('Origin',(32.85,3.0988,35.0707075174648));
#19689=CARTESIAN_POINT('',(32.85,3.0988,35.0707075174648));
#19690=CARTESIAN_POINT('Origin',(32.85,39.4248,20.95));
#19691=CARTESIAN_POINT('',(32.85,39.1748,20.7));
#19692=CARTESIAN_POINT('Origin',(32.85,39.4248,55.249));
#19693=CARTESIAN_POINT('',(32.85,39.1748,55.499));
#19694=CARTESIAN_POINT('Origin',(32.85,39.6748,55.499));
#19695=CARTESIAN_POINT('',(32.85,3.5988,55.499));
#19696=CARTESIAN_POINT('Origin',(32.85,3.3488,55.249));
#19697=CARTESIAN_POINT('',(32.85,3.0988,54.999));
#19698=CARTESIAN_POINT('Origin',(32.85,3.0988,55.499));
#19699=CARTESIAN_POINT('Origin',(32.85,19.4691107383531,20.7));
#71776=UNCERTAINTY_MEASURE_WITH_UNIT(LENGTH_MEASURE(0.01),#71796,
'DISTANCE_ACCURACY_VALUE',
'Maximum model space distance between geometric entities at asserted c
onnectivities');
#71783=UNCERTAINTY_MEASURE_WITH_UNIT(LENGTH_MEASURE(0.01),#71796,
'DISTANCE_ACCURACY_VALUE',
'Maximum model space distance between geometric entities at asserted c
onnectivities');
#71788=(
GEOMETRIC_REPRESENTATION_CONTEXT(3)
GLOBAL_UNCERTAINTY_ASSIGNED_CONTEXT((#71776))
GLOBAL_UNIT_ASSIGNED_CONTEXT((#71796,#71798,#71799))
REPRESENTATION_CONTEXT('','3D')
);
#71795=(
GEOMETRIC_REPRESENTATION_CONTEXT(3)
GLOBAL_UNCERTAINTY_ASSIGNED_CONTEXT((#71783))
GLOBAL_UNIT_ASSIGNED_CONTEXT((#71796,#71798,#71799))
REPRESENTATION_CONTEXT('','3D')
);
#71796=(
LENGTH_UNIT()
NAMED_UNIT(*)
SI_UNIT(.MILLI.,.METRE.)
);
#71798=(
NAMED_UNIT(*)
PLANE_ANGLE_UNIT()
SI_UNIT($,.RADIAN.)
);
#71799=(
NAMED_UNIT(*)
SI_UNIT($,.STERADIAN.)
SOLID_ANGLE_UNIT()
);
#71804=SHAPE_DEFINITION_REPRESENTATION(#71815,#72020);
#71815=PRODUCT_DEFINITION_SHAPE('',$,#72032);
#72020=SHAPE_REPRESENTATION('',(#14012),#71788);
#72027=PRODUCT_DEFINITION_CONTEXT('part definition',#72062,'design');
#72032=PRODUCT_DEFINITION('Open Pillow Block Bushing Housing',
'Open Pillow Block Bushing Housing',#72043,#72027);
#72043=PRODUCT_DEFINITION_FORMATION('',$,#72068);
#72062=APPLICATION_CONTEXT(
'Core Data for Automotive Mechanical Design Process');
#72063=PRODUCT_CONTEXT('part definition',#72062,'mechanical');
#72068=PRODUCT('Open Pillow Block Bushing Housing',
'Open Pillow Block Bushing Housing',$,(#72063));
#72079=PRESENTATION_STYLE_ASSIGNMENT((#72090));
#72090=SURFACE_STYLE_USAGE(.BOTH.,#72101);
#72101=SURFACE_SIDE_STYLE('',(#72112));
#72112=SURFACE_STYLE_FILL_AREA(#72123);
#72123=FILL_AREA_STYLE('Opaque(214,217,222)',(#72134));
#72134=FILL_AREA_STYLE_COLOUR('Opaque(214,217,222)',#72145);
#72145=COLOUR_RGB('Opaque(214,217,222)', 0.40784314, 0.44705882, 0.49803922);
ENDSEC;
END-ISO-10303-21;
